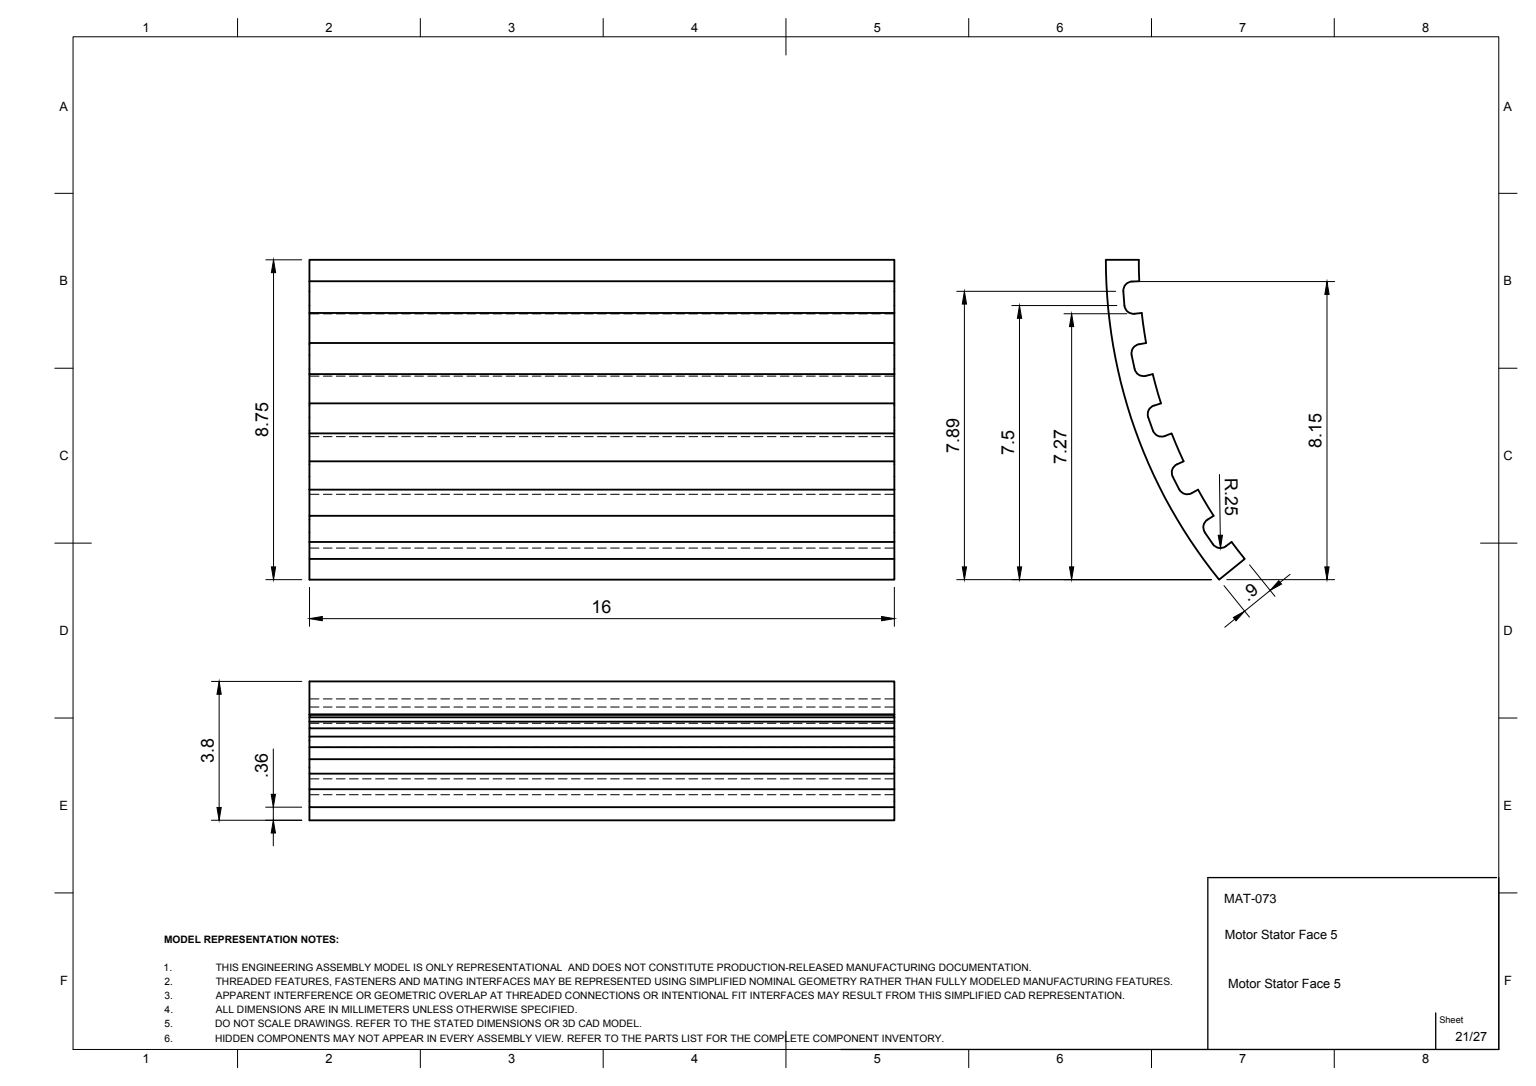
ISO-10303-21;
HEADER;
/* Generated by software containing ST-Developer
 * from STEP Tools, Inc. (www.steptools.com) 
 */

FILE_DESCRIPTION(
/* description */ ('CAx-IF Rec.Pracs.---Representation and Presentation of Product Manufa
cturing Information (PMI)---4.0---2014-10-13'),
/* implementation_level */ '2;1');

FILE_NAME(
/* name */ 'Motor Stator Face 5.step',
/* time_stamp */ '2026-10-24T18:52:33-07:00',
/* author */ (''),
/* organization */ (''),
/* preprocessor_version */ 'ST-DEVELOPER v20.2',
/* originating_system */ 'Autodesk Translation Framework v15.17.0.0',
/* authorisation */ '');

FILE_SCHEMA (('AP242_MANAGED_MODEL_BASED_3D_ENGINEERING_MIM_LF { 1 0 10303 442 2 1 4 }'));
ENDSEC;

DATA;
#10=MECHANICAL_DESIGN_GEOMETRIC_PRESENTATION_REPRESENTATION('',(#436),#34876);
#370=SHAPE_REPRESENTATION_RELATIONSHIP('SRR','None',#35007,#403);
#403=ADVANCED_BREP_SHAPE_REPRESENTATION('',(#469),#34865);
#436=STYLED_ITEM('',(#35165),#469);
#469=MANIFOLD_SOLID_BREP('Motor Stator Face 5',#19576);
#929=PLANE('',#21677);
#930=PLANE('',#21687);
#931=PLANE('',#21697);
#932=PLANE('',#21707);
#933=PLANE('',#21717);
#934=PLANE('',#21718);
#935=PLANE('',#21719);
#936=PLANE('',#21720);
#937=PLANE('',#21721);
#938=PLANE('',#21728);
#939=PLANE('',#21738);
#940=PLANE('',#21741);
#941=PLANE('',#21744);
#942=PLANE('',#21747);
#2176=LINE('',#32962,#3775);
#2177=LINE('',#32965,#3776);
#2178=LINE('',#32970,#3777);
#2179=LINE('',#32976,#3778);
#2180=LINE('',#32980,#3779);
#2181=LINE('',#32982,#3780);
#2182=LINE('',#32983,#3781);
#2183=LINE('',#32989,#3782);
#2184=LINE('',#32992,#3783);
#2185=LINE('',#32997,#3784);
#2186=LINE('',#33003,#3785);
#2187=LINE('',#33007,#3786);
#2188=LINE('',#33009,#3787);
#2189=LINE('',#33010,#3788);
#2190=LINE('',#33016,#3789);
#2191=LINE('',#33019,#3790);
#2192=LINE('',#33024,#3791);
#2193=LINE('',#33030,#3792);
#2194=LINE('',#33034,#3793);
#2195=LINE('',#33036,#3794);
#2196=LINE('',#33037,#3795);
#2197=LINE('',#33043,#3796);
#2198=LINE('',#33046,#3797);
#2199=LINE('',#33051,#3798);
#2200=LINE('',#33057,#3799);
#2201=LINE('',#33061,#3800);
#2202=LINE('',#33063,#3801);
#2203=LINE('',#33064,#3802);
#2204=LINE('',#33070,#3803);
#2205=LINE('',#33073,#3804);
#2206=LINE('',#33078,#3805);
#2207=LINE('',#33084,#3806);
#2208=LINE('',#33088,#3807);
#2209=LINE('',#33090,#3808);
#2210=LINE('',#33091,#3809);
#2211=LINE('',#33094,#3810);
#2212=LINE('',#33096,#3811);
#2213=LINE('',#33097,#3812);
#2214=LINE('',#33100,#3813);
#2215=LINE('',#33102,#3814);
#2216=LINE('',#33103,#3815);
#2217=LINE('',#33106,#3816);
#2218=LINE('',#33108,#3817);
#2219=LINE('',#33109,#3818);
#2220=LINE('',#33112,#3819);
#2221=LINE('',#33114,#3820);
#2222=LINE('',#33115,#3821);
#2223=LINE('',#33120,#3822);
#2224=LINE('',#33127,#3823);
#2225=LINE('',#33131,#3824);
#2226=LINE('',#33136,#3825);
#2227=LINE('',#33141,#3826);
#2228=LINE('',#33144,#3827);
#2229=LINE('',#33147,#3828);
#2230=LINE('',#33152,#3829);
#2231=LINE('',#33153,#3830);
#2232=LINE('',#33157,#3831);
#2233=LINE('',#33159,#3832);
#3775=VECTOR('',#26789,1.);
#3776=VECTOR('',#26792,1.);
#3777=VECTOR('',#26797,1.);
#3778=VECTOR('',#26804,1.);
#3779=VECTOR('',#26809,1.);
#3780=VECTOR('',#26810,1.);
#3781=VECTOR('',#26811,1.);
#3782=VECTOR('',#26816,1.);
#3783=VECTOR('',#26819,1.);
#3784=VECTOR('',#26824,1.);
#3785=VECTOR('',#26831,1.);
#3786=VECTOR('',#26836,1.);
#3787=VECTOR('',#26837,1.);
#3788=VECTOR('',#26838,1.);
#3789=VECTOR('',#26843,1.);
#3790=VECTOR('',#26846,1.);
#3791=VECTOR('',#26851,1.);
#3792=VECTOR('',#26858,1.);
#3793=VECTOR('',#26863,1.);
#3794=VECTOR('',#26864,1.);
#3795=VECTOR('',#26865,1.);
#3796=VECTOR('',#26870,1.);
#3797=VECTOR('',#26873,1.);
#3798=VECTOR('',#26878,1.);
#3799=VECTOR('',#26885,1.);
#3800=VECTOR('',#26890,1.);
#3801=VECTOR('',#26891,1.);
#3802=VECTOR('',#26892,1.);
#3803=VECTOR('',#26897,1.);
#3804=VECTOR('',#26900,1.);
#3805=VECTOR('',#26905,1.);
#3806=VECTOR('',#26912,1.);
#3807=VECTOR('',#26917,1.);
#3808=VECTOR('',#26918,1.);
#3809=VECTOR('',#26919,1.);
#3810=VECTOR('',#26922,1.);
#3811=VECTOR('',#26923,1.);
#3812=VECTOR('',#26924,1.);
#3813=VECTOR('',#26927,1.);
#3814=VECTOR('',#26928,1.);
#3815=VECTOR('',#26929,1.);
#3816=VECTOR('',#26932,1.);
#3817=VECTOR('',#26933,1.);
#3818=VECTOR('',#26934,1.);
#3819=VECTOR('',#26937,1.);
#3820=VECTOR('',#26938,1.);
#3821=VECTOR('',#26939,1.);
#3822=VECTOR('',#26944,1.);
#3823=VECTOR('',#26955,1.);
#3824=VECTOR('',#26958,1.);
#3825=VECTOR('',#26965,1.);
#3826=VECTOR('',#26972,1.);
#3827=VECTOR('',#26975,1.);
#3828=VECTOR('',#26980,1.);
#3829=VECTOR('',#26987,1.);
#3830=VECTOR('',#26988,1.);
#3831=VECTOR('',#26993,1.);
#3832=VECTOR('',#26996,1.);
#4681=CYLINDRICAL_SURFACE('',#21668,0.00025);
#4682=CYLINDRICAL_SURFACE('',#21671,0.01345);
#4683=CYLINDRICAL_SURFACE('',#21674,0.00025);
#4684=CYLINDRICAL_SURFACE('',#21678,0.00025);
#4685=CYLINDRICAL_SURFACE('',#21681,0.01345);
#4686=CYLINDRICAL_SURFACE('',#21684,0.00025);
#4687=CYLINDRICAL_SURFACE('',#21688,0.00025);
#4688=CYLINDRICAL_SURFACE('',#21691,0.01345);
#4689=CYLINDRICAL_SURFACE('',#21694,0.00025);
#4690=CYLINDRICAL_SURFACE('',#21698,0.00025);
#4691=CYLINDRICAL_SURFACE('',#21701,0.01345);
#4692=CYLINDRICAL_SURFACE('',#21704,0.00025);
#4693=CYLINDRICAL_SURFACE('',#21708,0.00025);
#4694=CYLINDRICAL_SURFACE('',#21711,0.01345);
#4695=CYLINDRICAL_SURFACE('',#21714,0.00025);
#4696=CYLINDRICAL_SURFACE('',#21722,0.013);
#4697=CYLINDRICAL_SURFACE('',#21725,0.013);
#4698=CYLINDRICAL_SURFACE('',#21734,0.013);
#4699=CYLINDRICAL_SURFACE('',#21736,0.013);
#4700=CYLINDRICAL_SURFACE('',#21739,0.013);
#4701=CYLINDRICAL_SURFACE('',#21742,0.0139);
#4702=CYLINDRICAL_SURFACE('',#21745,0.013);
#5552=FACE_OUTER_BOUND('',#6679,.T.);
#5553=FACE_OUTER_BOUND('',#6680,.T.);
#5554=FACE_OUTER_BOUND('',#6681,.T.);
#5555=FACE_OUTER_BOUND('',#6682,.T.);
#5556=FACE_OUTER_BOUND('',#6683,.T.);
#5557=FACE_OUTER_BOUND('',#6684,.T.);
#5558=FACE_OUTER_BOUND('',#6685,.T.);
#5559=FACE_OUTER_BOUND('',#6686,.T.);
#5560=FACE_OUTER_BOUND('',#6687,.T.);
#5561=FACE_OUTER_BOUND('',#6688,.T.);
#5562=FACE_OUTER_BOUND('',#6689,.T.);
#5563=FACE_OUTER_BOUND('',#6690,.T.);
#5564=FACE_OUTER_BOUND('',#6691,.T.);
#5565=FACE_OUTER_BOUND('',#6692,.T.);
#5566=FACE_OUTER_BOUND('',#6693,.T.);
#5567=FACE_OUTER_BOUND('',#6694,.T.);
#5568=FACE_OUTER_BOUND('',#6695,.T.);
#5569=FACE_OUTER_BOUND('',#6696,.T.);
#5570=FACE_OUTER_BOUND('',#6697,.T.);
#5571=FACE_OUTER_BOUND('',#6698,.T.);
#5572=FACE_OUTER_BOUND('',#6699,.T.);
#5573=FACE_OUTER_BOUND('',#6700,.T.);
#5574=FACE_OUTER_BOUND('',#6701,.T.);
#5575=FACE_OUTER_BOUND('',#6702,.T.);
#5576=FACE_OUTER_BOUND('',#6703,.T.);
#5577=FACE_OUTER_BOUND('',#6704,.T.);
#5578=FACE_OUTER_BOUND('',#6705,.T.);
#5579=FACE_OUTER_BOUND('',#6706,.T.);
#5580=FACE_OUTER_BOUND('',#6707,.T.);
#5581=FACE_OUTER_BOUND('',#6708,.T.);
#5582=FACE_OUTER_BOUND('',#6709,.T.);
#5583=FACE_OUTER_BOUND('',#6710,.T.);
#5584=FACE_OUTER_BOUND('',#6711,.T.);
#5585=FACE_OUTER_BOUND('',#6712,.T.);
#5586=FACE_OUTER_BOUND('',#6713,.T.);
#5587=FACE_OUTER_BOUND('',#6714,.T.);
#6679=EDGE_LOOP('',(#16904,#16905,#16906,#16907));
#6680=EDGE_LOOP('',(#16908,#16909,#16910,#16911));
#6681=EDGE_LOOP('',(#16912,#16913,#16914,#16915));
#6682=EDGE_LOOP('',(#16916,#16917,#16918,#16919));
#6683=EDGE_LOOP('',(#16920,#16921,#16922,#16923));
#6684=EDGE_LOOP('',(#16924,#16925,#16926,#16927));
#6685=EDGE_LOOP('',(#16928,#16929,#16930,#16931));
#6686=EDGE_LOOP('',(#16932,#16933,#16934,#16935));
#6687=EDGE_LOOP('',(#16936,#16937,#16938,#16939));
#6688=EDGE_LOOP('',(#16940,#16941,#16942,#16943));
#6689=EDGE_LOOP('',(#16944,#16945,#16946,#16947));
#6690=EDGE_LOOP('',(#16948,#16949,#16950,#16951));
#6691=EDGE_LOOP('',(#16952,#16953,#16954,#16955));
#6692=EDGE_LOOP('',(#16956,#16957,#16958,#16959));
#6693=EDGE_LOOP('',(#16960,#16961,#16962,#16963));
#6694=EDGE_LOOP('',(#16964,#16965,#16966,#16967));
#6695=EDGE_LOOP('',(#16968,#16969,#16970,#16971));
#6696=EDGE_LOOP('',(#16972,#16973,#16974,#16975));
#6697=EDGE_LOOP('',(#16976,#16977,#16978,#16979));
#6698=EDGE_LOOP('',(#16980,#16981,#16982,#16983));
#6699=EDGE_LOOP('',(#16984,#16985,#16986,#16987));
#6700=EDGE_LOOP('',(#16988,#16989,#16990,#16991));
#6701=EDGE_LOOP('',(#16992,#16993,#16994,#16995));
#6702=EDGE_LOOP('',(#16996,#16997,#16998,#16999));
#6703=EDGE_LOOP('',(#17000,#17001,#17002,#17003));
#6704=EDGE_LOOP('',(#17004,#17005,#17006,#17007));
#6705=EDGE_LOOP('',(#17008,#17009,#17010,#17011,#17012,#17013,#17014,#17015,
#17016,#17017,#17018,#17019,#17020,#17021,#17022,#17023,#17024,#17025,#17026,
#17027,#17028,#17029,#17030,#17031,#17032,#17033,#17034,#17035,#17036,#17037,
#17038,#17039,#17040,#17041));
#6706=EDGE_LOOP('',(#17042,#17043,#17044,#17045));
#6707=EDGE_LOOP('',(#17046,#17047,#17048,#17049));
#6708=EDGE_LOOP('',(#17050,#17051,#17052,#17053));
#6709=EDGE_LOOP('',(#17054,#17055,#17056,#17057));
#6710=EDGE_LOOP('',(#17058,#17059,#17060,#17061));
#6711=EDGE_LOOP('',(#17062,#17063,#17064,#17065));
#6712=EDGE_LOOP('',(#17066,#17067,#17068,#17069));
#6713=EDGE_LOOP('',(#17070,#17071,#17072,#17073));
#6714=EDGE_LOOP('',(#17074,#17075,#17076,#17077,#17078,#17079,#17080,#17081,
#17082,#17083,#17084,#17085,#17086,#17087,#17088,#17089,#17090,#17091,#17092,
#17093,#17094,#17095,#17096,#17097,#17098,#17099,#17100,#17101,#17102,#17103,
#17104,#17105,#17106,#17107));
#7815=CIRCLE('',#21669,0.000250000000013569);
#7816=CIRCLE('',#21670,0.000250000000013569);
#7817=CIRCLE('',#21672,0.0134500000000125);
#7818=CIRCLE('',#21673,0.0134500000000125);
#7819=CIRCLE('',#21675,0.000250000000013744);
#7820=CIRCLE('',#21676,0.000250000000013744);
#7821=CIRCLE('',#21679,0.000250000000013973);
#7822=CIRCLE('',#21680,0.000250000000013973);
#7823=CIRCLE('',#21682,0.0134500000000115);
#7824=CIRCLE('',#21683,0.0134500000000115);
#7825=CIRCLE('',#21685,0.000250000000014062);
#7826=CIRCLE('',#21686,0.000250000000014062);
#7827=CIRCLE('',#21689,0.000250000000014138);
#7828=CIRCLE('',#21690,0.000250000000014138);
#7829=CIRCLE('',#21692,0.0134500000000103);
#7830=CIRCLE('',#21693,0.0134500000000103);
#7831=CIRCLE('',#21695,0.000250000000014138);
#7832=CIRCLE('',#21696,0.000250000000014138);
#7833=CIRCLE('',#21699,0.000250000000014062);
#7834=CIRCLE('',#21700,0.000250000000014062);
#7835=CIRCLE('',#21702,0.0134500000000109);
#7836=CIRCLE('',#21703,0.0134500000000109);
#7837=CIRCLE('',#21705,0.000250000000013973);
#7838=CIRCLE('',#21706,0.000250000000013973);
#7839=CIRCLE('',#21709,0.000250000000013744);
#7840=CIRCLE('',#21710,0.000250000000013744);
#7841=CIRCLE('',#21712,0.013450000000012);
#7842=CIRCLE('',#21713,0.013450000000012);
#7843=CIRCLE('',#21715,0.000250000000013569);
#7844=CIRCLE('',#21716,0.000250000000013569);
#7845=CIRCLE('',#21723,0.0130000000000128);
#7846=CIRCLE('',#21724,0.0130000000000128);
#7847=CIRCLE('',#21726,0.0130000000000128);
#7848=CIRCLE('',#21727,0.0130000000000128);
#7849=CIRCLE('',#21729,0.0139000000000128);
#7850=CIRCLE('',#21730,0.0130000000000128);
#7851=CIRCLE('',#21731,0.0130000000000128);
#7852=CIRCLE('',#21732,0.0130000000000128);
#7853=CIRCLE('',#21733,0.0130000000000128);
#7854=CIRCLE('',#21735,0.0130000000000128);
#7855=CIRCLE('',#21737,0.0130000000000128);
#7856=CIRCLE('',#21740,0.0130000000000128);
#7857=CIRCLE('',#21743,0.0139000000000128);
#7858=CIRCLE('',#21746,0.0130000000000128);
#9431=VERTEX_POINT('',#32958);
#9432=VERTEX_POINT('',#32959);
#9433=VERTEX_POINT('',#32961);
#9434=VERTEX_POINT('',#32963);
#9435=VERTEX_POINT('',#32967);
#9436=VERTEX_POINT('',#32969);
#9437=VERTEX_POINT('',#32973);
#9438=VERTEX_POINT('',#32975);
#9439=VERTEX_POINT('',#32979);
#9440=VERTEX_POINT('',#32981);
#9441=VERTEX_POINT('',#32985);
#9442=VERTEX_POINT('',#32986);
#9443=VERTEX_POINT('',#32988);
#9444=VERTEX_POINT('',#32990);
#9445=VERTEX_POINT('',#32994);
#9446=VERTEX_POINT('',#32996);
#9447=VERTEX_POINT('',#33000);
#9448=VERTEX_POINT('',#33002);
#9449=VERTEX_POINT('',#33006);
#9450=VERTEX_POINT('',#33008);
#9451=VERTEX_POINT('',#33012);
#9452=VERTEX_POINT('',#33013);
#9453=VERTEX_POINT('',#33015);
#9454=VERTEX_POINT('',#33017);
#9455=VERTEX_POINT('',#33021);
#9456=VERTEX_POINT('',#33023);
#9457=VERTEX_POINT('',#33027);
#9458=VERTEX_POINT('',#33029);
#9459=VERTEX_POINT('',#33033);
#9460=VERTEX_POINT('',#33035);
#9461=VERTEX_POINT('',#33039);
#9462=VERTEX_POINT('',#33040);
#9463=VERTEX_POINT('',#33042);
#9464=VERTEX_POINT('',#33044);
#9465=VERTEX_POINT('',#33048);
#9466=VERTEX_POINT('',#33050);
#9467=VERTEX_POINT('',#33054);
#9468=VERTEX_POINT('',#33056);
#9469=VERTEX_POINT('',#33060);
#9470=VERTEX_POINT('',#33062);
#9471=VERTEX_POINT('',#33066);
#9472=VERTEX_POINT('',#33067);
#9473=VERTEX_POINT('',#33069);
#9474=VERTEX_POINT('',#33071);
#9475=VERTEX_POINT('',#33075);
#9476=VERTEX_POINT('',#33077);
#9477=VERTEX_POINT('',#33081);
#9478=VERTEX_POINT('',#33083);
#9479=VERTEX_POINT('',#33087);
#9480=VERTEX_POINT('',#33089);
#9481=VERTEX_POINT('',#33093);
#9482=VERTEX_POINT('',#33095);
#9483=VERTEX_POINT('',#33099);
#9484=VERTEX_POINT('',#33101);
#9485=VERTEX_POINT('',#33105);
#9486=VERTEX_POINT('',#33107);
#9487=VERTEX_POINT('',#33111);
#9488=VERTEX_POINT('',#33113);
#9489=VERTEX_POINT('',#33117);
#9490=VERTEX_POINT('',#33119);
#9491=VERTEX_POINT('',#33126);
#9492=VERTEX_POINT('',#33128);
#9493=VERTEX_POINT('',#33130);
#9494=VERTEX_POINT('',#33134);
#9495=VERTEX_POINT('',#33139);
#9496=VERTEX_POINT('',#33143);
#9497=VERTEX_POINT('',#33151);
#9498=VERTEX_POINT('',#33155);
#12010=EDGE_CURVE('',#9431,#9432,#7815,.T.);
#12011=EDGE_CURVE('',#9432,#9433,#2176,.T.);
#12012=EDGE_CURVE('',#9433,#9434,#7816,.T.);
#12013=EDGE_CURVE('',#9434,#9431,#2177,.T.);
#12014=EDGE_CURVE('',#9435,#9432,#7817,.T.);
#12015=EDGE_CURVE('',#9436,#9435,#2178,.T.);
#12016=EDGE_CURVE('',#9433,#9436,#7818,.T.);
#12017=EDGE_CURVE('',#9435,#9437,#7819,.T.);
#12018=EDGE_CURVE('',#9437,#9438,#2179,.T.);
#12019=EDGE_CURVE('',#9438,#9436,#7820,.T.);
#12020=EDGE_CURVE('',#9439,#9437,#2180,.T.);
#12021=EDGE_CURVE('',#9440,#9439,#2181,.T.);
#12022=EDGE_CURVE('',#9438,#9440,#2182,.T.);
#12023=EDGE_CURVE('',#9441,#9442,#7821,.T.);
#12024=EDGE_CURVE('',#9442,#9443,#2183,.T.);
#12025=EDGE_CURVE('',#9443,#9444,#7822,.T.);
#12026=EDGE_CURVE('',#9444,#9441,#2184,.T.);
#12027=EDGE_CURVE('',#9445,#9442,#7823,.T.);
#12028=EDGE_CURVE('',#9446,#9445,#2185,.T.);
#12029=EDGE_CURVE('',#9443,#9446,#7824,.T.);
#12030=EDGE_CURVE('',#9445,#9447,#7825,.T.);
#12031=EDGE_CURVE('',#9447,#9448,#2186,.T.);
#12032=EDGE_CURVE('',#9448,#9446,#7826,.T.);
#12033=EDGE_CURVE('',#9449,#9447,#2187,.T.);
#12034=EDGE_CURVE('',#9450,#9449,#2188,.T.);
#12035=EDGE_CURVE('',#9448,#9450,#2189,.T.);
#12036=EDGE_CURVE('',#9451,#9452,#7827,.T.);
#12037=EDGE_CURVE('',#9452,#9453,#2190,.T.);
#12038=EDGE_CURVE('',#9453,#9454,#7828,.T.);
#12039=EDGE_CURVE('',#9454,#9451,#2191,.T.);
#12040=EDGE_CURVE('',#9455,#9452,#7829,.T.);
#12041=EDGE_CURVE('',#9456,#9455,#2192,.T.);
#12042=EDGE_CURVE('',#9453,#9456,#7830,.T.);
#12043=EDGE_CURVE('',#9455,#9457,#7831,.T.);
#12044=EDGE_CURVE('',#9457,#9458,#2193,.T.);
#12045=EDGE_CURVE('',#9458,#9456,#7832,.T.);
#12046=EDGE_CURVE('',#9459,#9457,#2194,.T.);
#12047=EDGE_CURVE('',#9460,#9459,#2195,.T.);
#12048=EDGE_CURVE('',#9458,#9460,#2196,.T.);
#12049=EDGE_CURVE('',#9461,#9462,#7833,.T.);
#12050=EDGE_CURVE('',#9462,#9463,#2197,.T.);
#12051=EDGE_CURVE('',#9463,#9464,#7834,.T.);
#12052=EDGE_CURVE('',#9464,#9461,#2198,.T.);
#12053=EDGE_CURVE('',#9465,#9462,#7835,.T.);
#12054=EDGE_CURVE('',#9466,#9465,#2199,.T.);
#12055=EDGE_CURVE('',#9463,#9466,#7836,.T.);
#12056=EDGE_CURVE('',#9465,#9467,#7837,.T.);
#12057=EDGE_CURVE('',#9467,#9468,#2200,.T.);
#12058=EDGE_CURVE('',#9468,#9466,#7838,.T.);
#12059=EDGE_CURVE('',#9469,#9467,#2201,.T.);
#12060=EDGE_CURVE('',#9470,#9469,#2202,.T.);
#12061=EDGE_CURVE('',#9468,#9470,#2203,.T.);
#12062=EDGE_CURVE('',#9471,#9472,#7839,.T.);
#12063=EDGE_CURVE('',#9472,#9473,#2204,.T.);
#12064=EDGE_CURVE('',#9473,#9474,#7840,.T.);
#12065=EDGE_CURVE('',#9474,#9471,#2205,.T.);
#12066=EDGE_CURVE('',#9475,#9472,#7841,.T.);
#12067=EDGE_CURVE('',#9476,#9475,#2206,.T.);
#12068=EDGE_CURVE('',#9473,#9476,#7842,.T.);
#12069=EDGE_CURVE('',#9475,#9477,#7843,.T.);
#12070=EDGE_CURVE('',#9477,#9478,#2207,.T.);
#12071=EDGE_CURVE('',#9478,#9476,#7844,.T.);
#12072=EDGE_CURVE('',#9479,#9477,#2208,.T.);
#12073=EDGE_CURVE('',#9480,#9479,#2209,.T.);
#12074=EDGE_CURVE('',#9478,#9480,#2210,.T.);
#12075=EDGE_CURVE('',#9481,#9474,#2211,.T.);
#12076=EDGE_CURVE('',#9482,#9481,#2212,.T.);
#12077=EDGE_CURVE('',#9471,#9482,#2213,.T.);
#12078=EDGE_CURVE('',#9483,#9464,#2214,.T.);
#12079=EDGE_CURVE('',#9484,#9483,#2215,.T.);
#12080=EDGE_CURVE('',#9461,#9484,#2216,.T.);
#12081=EDGE_CURVE('',#9485,#9444,#2217,.T.);
#12082=EDGE_CURVE('',#9486,#9485,#2218,.T.);
#12083=EDGE_CURVE('',#9441,#9486,#2219,.T.);
#12084=EDGE_CURVE('',#9487,#9434,#2220,.T.);
#12085=EDGE_CURVE('',#9488,#9487,#2221,.T.);
#12086=EDGE_CURVE('',#9431,#9488,#2222,.T.);
#12087=EDGE_CURVE('',#9489,#9479,#7845,.T.);
#12088=EDGE_CURVE('',#9489,#9490,#2223,.T.);
#12089=EDGE_CURVE('',#9480,#9490,#7846,.T.);
#12090=EDGE_CURVE('',#9460,#9483,#7847,.T.);
#12091=EDGE_CURVE('',#9484,#9459,#7848,.T.);
#12092=EDGE_CURVE('',#9490,#9491,#2224,.T.);
#12093=EDGE_CURVE('',#9491,#9492,#7849,.T.);
#12094=EDGE_CURVE('',#9492,#9493,#2225,.T.);
#12095=EDGE_CURVE('',#9493,#9487,#7850,.T.);
#12096=EDGE_CURVE('',#9440,#9485,#7851,.T.);
#12097=EDGE_CURVE('',#9450,#9494,#7852,.T.);
#12098=EDGE_CURVE('',#9494,#9454,#2226,.T.);
#12099=EDGE_CURVE('',#9470,#9481,#7853,.T.);
#12100=EDGE_CURVE('',#9495,#9449,#7854,.T.);
#12101=EDGE_CURVE('',#9495,#9494,#2227,.T.);
#12102=EDGE_CURVE('',#9493,#9496,#2228,.T.);
#12103=EDGE_CURVE('',#9488,#9496,#7855,.T.);
#12104=EDGE_CURVE('',#9451,#9495,#2229,.T.);
#12105=EDGE_CURVE('',#9482,#9469,#7856,.T.);
#12106=EDGE_CURVE('',#9497,#9489,#2230,.T.);
#12107=EDGE_CURVE('',#9491,#9497,#2231,.T.);
#12108=EDGE_CURVE('',#9498,#9497,#7857,.T.);
#12109=EDGE_CURVE('',#9492,#9498,#2232,.T.);
#12110=EDGE_CURVE('',#9496,#9498,#2233,.T.);
#12111=EDGE_CURVE('',#9486,#9439,#7858,.T.);
#16904=ORIENTED_EDGE('',*,*,#12010,.T.);
#16905=ORIENTED_EDGE('',*,*,#12011,.T.);
#16906=ORIENTED_EDGE('',*,*,#12012,.T.);
#16907=ORIENTED_EDGE('',*,*,#12013,.T.);
#16908=ORIENTED_EDGE('',*,*,#12011,.F.);
#16909=ORIENTED_EDGE('',*,*,#12014,.F.);
#16910=ORIENTED_EDGE('',*,*,#12015,.F.);
#16911=ORIENTED_EDGE('',*,*,#12016,.F.);
#16912=ORIENTED_EDGE('',*,*,#12017,.T.);
#16913=ORIENTED_EDGE('',*,*,#12018,.T.);
#16914=ORIENTED_EDGE('',*,*,#12019,.T.);
#16915=ORIENTED_EDGE('',*,*,#12015,.T.);
#16916=ORIENTED_EDGE('',*,*,#12018,.F.);
#16917=ORIENTED_EDGE('',*,*,#12020,.F.);
#16918=ORIENTED_EDGE('',*,*,#12021,.F.);
#16919=ORIENTED_EDGE('',*,*,#12022,.F.);
#16920=ORIENTED_EDGE('',*,*,#12023,.T.);
#16921=ORIENTED_EDGE('',*,*,#12024,.T.);
#16922=ORIENTED_EDGE('',*,*,#12025,.T.);
#16923=ORIENTED_EDGE('',*,*,#12026,.T.);
#16924=ORIENTED_EDGE('',*,*,#12024,.F.);
#16925=ORIENTED_EDGE('',*,*,#12027,.F.);
#16926=ORIENTED_EDGE('',*,*,#12028,.F.);
#16927=ORIENTED_EDGE('',*,*,#12029,.F.);
#16928=ORIENTED_EDGE('',*,*,#12030,.T.);
#16929=ORIENTED_EDGE('',*,*,#12031,.T.);
#16930=ORIENTED_EDGE('',*,*,#12032,.T.);
#16931=ORIENTED_EDGE('',*,*,#12028,.T.);
#16932=ORIENTED_EDGE('',*,*,#12031,.F.);
#16933=ORIENTED_EDGE('',*,*,#12033,.F.);
#16934=ORIENTED_EDGE('',*,*,#12034,.F.);
#16935=ORIENTED_EDGE('',*,*,#12035,.F.);
#16936=ORIENTED_EDGE('',*,*,#12036,.T.);
#16937=ORIENTED_EDGE('',*,*,#12037,.T.);
#16938=ORIENTED_EDGE('',*,*,#12038,.T.);
#16939=ORIENTED_EDGE('',*,*,#12039,.T.);
#16940=ORIENTED_EDGE('',*,*,#12037,.F.);
#16941=ORIENTED_EDGE('',*,*,#12040,.F.);
#16942=ORIENTED_EDGE('',*,*,#12041,.F.);
#16943=ORIENTED_EDGE('',*,*,#12042,.F.);
#16944=ORIENTED_EDGE('',*,*,#12043,.T.);
#16945=ORIENTED_EDGE('',*,*,#12044,.T.);
#16946=ORIENTED_EDGE('',*,*,#12045,.T.);
#16947=ORIENTED_EDGE('',*,*,#12041,.T.);
#16948=ORIENTED_EDGE('',*,*,#12044,.F.);
#16949=ORIENTED_EDGE('',*,*,#12046,.F.);
#16950=ORIENTED_EDGE('',*,*,#12047,.F.);
#16951=ORIENTED_EDGE('',*,*,#12048,.F.);
#16952=ORIENTED_EDGE('',*,*,#12049,.T.);
#16953=ORIENTED_EDGE('',*,*,#12050,.T.);
#16954=ORIENTED_EDGE('',*,*,#12051,.T.);
#16955=ORIENTED_EDGE('',*,*,#12052,.T.);
#16956=ORIENTED_EDGE('',*,*,#12050,.F.);
#16957=ORIENTED_EDGE('',*,*,#12053,.F.);
#16958=ORIENTED_EDGE('',*,*,#12054,.F.);
#16959=ORIENTED_EDGE('',*,*,#12055,.F.);
#16960=ORIENTED_EDGE('',*,*,#12056,.T.);
#16961=ORIENTED_EDGE('',*,*,#12057,.T.);
#16962=ORIENTED_EDGE('',*,*,#12058,.T.);
#16963=ORIENTED_EDGE('',*,*,#12054,.T.);
#16964=ORIENTED_EDGE('',*,*,#12057,.F.);
#16965=ORIENTED_EDGE('',*,*,#12059,.F.);
#16966=ORIENTED_EDGE('',*,*,#12060,.F.);
#16967=ORIENTED_EDGE('',*,*,#12061,.F.);
#16968=ORIENTED_EDGE('',*,*,#12062,.T.);
#16969=ORIENTED_EDGE('',*,*,#12063,.T.);
#16970=ORIENTED_EDGE('',*,*,#12064,.T.);
#16971=ORIENTED_EDGE('',*,*,#12065,.T.);
#16972=ORIENTED_EDGE('',*,*,#12063,.F.);
#16973=ORIENTED_EDGE('',*,*,#12066,.F.);
#16974=ORIENTED_EDGE('',*,*,#12067,.F.);
#16975=ORIENTED_EDGE('',*,*,#12068,.F.);
#16976=ORIENTED_EDGE('',*,*,#12069,.T.);
#16977=ORIENTED_EDGE('',*,*,#12070,.T.);
#16978=ORIENTED_EDGE('',*,*,#12071,.T.);
#16979=ORIENTED_EDGE('',*,*,#12067,.T.);
#16980=ORIENTED_EDGE('',*,*,#12070,.F.);
#16981=ORIENTED_EDGE('',*,*,#12072,.F.);
#16982=ORIENTED_EDGE('',*,*,#12073,.F.);
#16983=ORIENTED_EDGE('',*,*,#12074,.F.);
#16984=ORIENTED_EDGE('',*,*,#12065,.F.);
#16985=ORIENTED_EDGE('',*,*,#12075,.F.);
#16986=ORIENTED_EDGE('',*,*,#12076,.F.);
#16987=ORIENTED_EDGE('',*,*,#12077,.F.);
#16988=ORIENTED_EDGE('',*,*,#12052,.F.);
#16989=ORIENTED_EDGE('',*,*,#12078,.F.);
#16990=ORIENTED_EDGE('',*,*,#12079,.F.);
#16991=ORIENTED_EDGE('',*,*,#12080,.F.);
#16992=ORIENTED_EDGE('',*,*,#12026,.F.);
#16993=ORIENTED_EDGE('',*,*,#12081,.F.);
#16994=ORIENTED_EDGE('',*,*,#12082,.F.);
#16995=ORIENTED_EDGE('',*,*,#12083,.F.);
#16996=ORIENTED_EDGE('',*,*,#12013,.F.);
#16997=ORIENTED_EDGE('',*,*,#12084,.F.);
#16998=ORIENTED_EDGE('',*,*,#12085,.F.);
#16999=ORIENTED_EDGE('',*,*,#12086,.F.);
#17000=ORIENTED_EDGE('',*,*,#12073,.T.);
#17001=ORIENTED_EDGE('',*,*,#12087,.F.);
#17002=ORIENTED_EDGE('',*,*,#12088,.T.);
#17003=ORIENTED_EDGE('',*,*,#12089,.F.);
#17004=ORIENTED_EDGE('',*,*,#12079,.T.);
#17005=ORIENTED_EDGE('',*,*,#12090,.F.);
#17006=ORIENTED_EDGE('',*,*,#12047,.T.);
#17007=ORIENTED_EDGE('',*,*,#12091,.F.);
#17008=ORIENTED_EDGE('',*,*,#12075,.T.);
#17009=ORIENTED_EDGE('',*,*,#12064,.F.);
#17010=ORIENTED_EDGE('',*,*,#12068,.T.);
#17011=ORIENTED_EDGE('',*,*,#12071,.F.);
#17012=ORIENTED_EDGE('',*,*,#12074,.T.);
#17013=ORIENTED_EDGE('',*,*,#12089,.T.);
#17014=ORIENTED_EDGE('',*,*,#12092,.T.);
#17015=ORIENTED_EDGE('',*,*,#12093,.T.);
#17016=ORIENTED_EDGE('',*,*,#12094,.T.);
#17017=ORIENTED_EDGE('',*,*,#12095,.T.);
#17018=ORIENTED_EDGE('',*,*,#12084,.T.);
#17019=ORIENTED_EDGE('',*,*,#12012,.F.);
#17020=ORIENTED_EDGE('',*,*,#12016,.T.);
#17021=ORIENTED_EDGE('',*,*,#12019,.F.);
#17022=ORIENTED_EDGE('',*,*,#12022,.T.);
#17023=ORIENTED_EDGE('',*,*,#12096,.T.);
#17024=ORIENTED_EDGE('',*,*,#12081,.T.);
#17025=ORIENTED_EDGE('',*,*,#12025,.F.);
#17026=ORIENTED_EDGE('',*,*,#12029,.T.);
#17027=ORIENTED_EDGE('',*,*,#12032,.F.);
#17028=ORIENTED_EDGE('',*,*,#12035,.T.);
#17029=ORIENTED_EDGE('',*,*,#12097,.T.);
#17030=ORIENTED_EDGE('',*,*,#12098,.T.);
#17031=ORIENTED_EDGE('',*,*,#12038,.F.);
#17032=ORIENTED_EDGE('',*,*,#12042,.T.);
#17033=ORIENTED_EDGE('',*,*,#12045,.F.);
#17034=ORIENTED_EDGE('',*,*,#12048,.T.);
#17035=ORIENTED_EDGE('',*,*,#12090,.T.);
#17036=ORIENTED_EDGE('',*,*,#12078,.T.);
#17037=ORIENTED_EDGE('',*,*,#12051,.F.);
#17038=ORIENTED_EDGE('',*,*,#12055,.T.);
#17039=ORIENTED_EDGE('',*,*,#12058,.F.);
#17040=ORIENTED_EDGE('',*,*,#12061,.T.);
#17041=ORIENTED_EDGE('',*,*,#12099,.T.);
#17042=ORIENTED_EDGE('',*,*,#12034,.T.);
#17043=ORIENTED_EDGE('',*,*,#12100,.F.);
#17044=ORIENTED_EDGE('',*,*,#12101,.T.);
#17045=ORIENTED_EDGE('',*,*,#12097,.F.);
#17046=ORIENTED_EDGE('',*,*,#12085,.T.);
#17047=ORIENTED_EDGE('',*,*,#12095,.F.);
#17048=ORIENTED_EDGE('',*,*,#12102,.T.);
#17049=ORIENTED_EDGE('',*,*,#12103,.F.);
#17050=ORIENTED_EDGE('',*,*,#12039,.F.);
#17051=ORIENTED_EDGE('',*,*,#12098,.F.);
#17052=ORIENTED_EDGE('',*,*,#12101,.F.);
#17053=ORIENTED_EDGE('',*,*,#12104,.F.);
#17054=ORIENTED_EDGE('',*,*,#12076,.T.);
#17055=ORIENTED_EDGE('',*,*,#12099,.F.);
#17056=ORIENTED_EDGE('',*,*,#12060,.T.);
#17057=ORIENTED_EDGE('',*,*,#12105,.F.);
#17058=ORIENTED_EDGE('',*,*,#12088,.F.);
#17059=ORIENTED_EDGE('',*,*,#12106,.F.);
#17060=ORIENTED_EDGE('',*,*,#12107,.F.);
#17061=ORIENTED_EDGE('',*,*,#12092,.F.);
#17062=ORIENTED_EDGE('',*,*,#12107,.T.);
#17063=ORIENTED_EDGE('',*,*,#12108,.F.);
#17064=ORIENTED_EDGE('',*,*,#12109,.F.);
#17065=ORIENTED_EDGE('',*,*,#12093,.F.);
#17066=ORIENTED_EDGE('',*,*,#12109,.T.);
#17067=ORIENTED_EDGE('',*,*,#12110,.F.);
#17068=ORIENTED_EDGE('',*,*,#12102,.F.);
#17069=ORIENTED_EDGE('',*,*,#12094,.F.);
#17070=ORIENTED_EDGE('',*,*,#12082,.T.);
#17071=ORIENTED_EDGE('',*,*,#12096,.F.);
#17072=ORIENTED_EDGE('',*,*,#12021,.T.);
#17073=ORIENTED_EDGE('',*,*,#12111,.F.);
#17074=ORIENTED_EDGE('',*,*,#12077,.T.);
#17075=ORIENTED_EDGE('',*,*,#12105,.T.);
#17076=ORIENTED_EDGE('',*,*,#12059,.T.);
#17077=ORIENTED_EDGE('',*,*,#12056,.F.);
#17078=ORIENTED_EDGE('',*,*,#12053,.T.);
#17079=ORIENTED_EDGE('',*,*,#12049,.F.);
#17080=ORIENTED_EDGE('',*,*,#12080,.T.);
#17081=ORIENTED_EDGE('',*,*,#12091,.T.);
#17082=ORIENTED_EDGE('',*,*,#12046,.T.);
#17083=ORIENTED_EDGE('',*,*,#12043,.F.);
#17084=ORIENTED_EDGE('',*,*,#12040,.T.);
#17085=ORIENTED_EDGE('',*,*,#12036,.F.);
#17086=ORIENTED_EDGE('',*,*,#12104,.T.);
#17087=ORIENTED_EDGE('',*,*,#12100,.T.);
#17088=ORIENTED_EDGE('',*,*,#12033,.T.);
#17089=ORIENTED_EDGE('',*,*,#12030,.F.);
#17090=ORIENTED_EDGE('',*,*,#12027,.T.);
#17091=ORIENTED_EDGE('',*,*,#12023,.F.);
#17092=ORIENTED_EDGE('',*,*,#12083,.T.);
#17093=ORIENTED_EDGE('',*,*,#12111,.T.);
#17094=ORIENTED_EDGE('',*,*,#12020,.T.);
#17095=ORIENTED_EDGE('',*,*,#12017,.F.);
#17096=ORIENTED_EDGE('',*,*,#12014,.T.);
#17097=ORIENTED_EDGE('',*,*,#12010,.F.);
#17098=ORIENTED_EDGE('',*,*,#12086,.T.);
#17099=ORIENTED_EDGE('',*,*,#12103,.T.);
#17100=ORIENTED_EDGE('',*,*,#12110,.T.);
#17101=ORIENTED_EDGE('',*,*,#12108,.T.);
#17102=ORIENTED_EDGE('',*,*,#12106,.T.);
#17103=ORIENTED_EDGE('',*,*,#12087,.T.);
#17104=ORIENTED_EDGE('',*,*,#12072,.T.);
#17105=ORIENTED_EDGE('',*,*,#12069,.F.);
#17106=ORIENTED_EDGE('',*,*,#12066,.T.);
#17107=ORIENTED_EDGE('',*,*,#12062,.F.);
#19268=ADVANCED_FACE('',(#5552),#4681,.F.);
#19269=ADVANCED_FACE('',(#5553),#4682,.F.);
#19270=ADVANCED_FACE('',(#5554),#4683,.F.);
#19271=ADVANCED_FACE('',(#5555),#929,.F.);
#19272=ADVANCED_FACE('',(#5556),#4684,.F.);
#19273=ADVANCED_FACE('',(#5557),#4685,.F.);
#19274=ADVANCED_FACE('',(#5558),#4686,.F.);
#19275=ADVANCED_FACE('',(#5559),#930,.F.);
#19276=ADVANCED_FACE('',(#5560),#4687,.F.);
#19277=ADVANCED_FACE('',(#5561),#4688,.F.);
#19278=ADVANCED_FACE('',(#5562),#4689,.F.);
#19279=ADVANCED_FACE('',(#5563),#931,.F.);
#19280=ADVANCED_FACE('',(#5564),#4690,.F.);
#19281=ADVANCED_FACE('',(#5565),#4691,.F.);
#19282=ADVANCED_FACE('',(#5566),#4692,.F.);
#19283=ADVANCED_FACE('',(#5567),#932,.F.);
#19284=ADVANCED_FACE('',(#5568),#4693,.F.);
#19285=ADVANCED_FACE('',(#5569),#4694,.F.);
#19286=ADVANCED_FACE('',(#5570),#4695,.F.);
#19287=ADVANCED_FACE('',(#5571),#933,.F.);
#19288=ADVANCED_FACE('',(#5572),#934,.F.);
#19289=ADVANCED_FACE('',(#5573),#935,.F.);
#19290=ADVANCED_FACE('',(#5574),#936,.F.);
#19291=ADVANCED_FACE('',(#5575),#937,.F.);
#19292=ADVANCED_FACE('',(#5576),#4696,.F.);
#19293=ADVANCED_FACE('',(#5577),#4697,.F.);
#19294=ADVANCED_FACE('',(#5578),#938,.F.);
#19295=ADVANCED_FACE('',(#5579),#4698,.F.);
#19296=ADVANCED_FACE('',(#5580),#4699,.F.);
#19297=ADVANCED_FACE('',(#5581),#939,.F.);
#19298=ADVANCED_FACE('',(#5582),#4700,.F.);
#19299=ADVANCED_FACE('',(#5583),#940,.T.);
#19300=ADVANCED_FACE('',(#5584),#4701,.T.);
#19301=ADVANCED_FACE('',(#5585),#941,.T.);
#19302=ADVANCED_FACE('',(#5586),#4702,.F.);
#19303=ADVANCED_FACE('',(#5587),#942,.T.);
#19576=CLOSED_SHELL('',(#19268,#19269,#19270,#19271,#19272,#19273,#19274,
#19275,#19276,#19277,#19278,#19279,#19280,#19281,#19282,#19283,#19284,#19285,
#19286,#19287,#19288,#19289,#19290,#19291,#19292,#19293,#19294,#19295,#19296,
#19297,#19298,#19299,#19300,#19301,#19302,#19303));
#21667=AXIS2_PLACEMENT_3D('',#32956,#26783,#26784);
#21668=AXIS2_PLACEMENT_3D('',#32957,#26785,#26786);
#21669=AXIS2_PLACEMENT_3D('',#32960,#26787,#26788);
#21670=AXIS2_PLACEMENT_3D('',#32964,#26790,#26791);
#21671=AXIS2_PLACEMENT_3D('',#32966,#26793,#26794);
#21672=AXIS2_PLACEMENT_3D('',#32968,#26795,#26796);
#21673=AXIS2_PLACEMENT_3D('',#32971,#26798,#26799);
#21674=AXIS2_PLACEMENT_3D('',#32972,#26800,#26801);
#21675=AXIS2_PLACEMENT_3D('',#32974,#26802,#26803);
#21676=AXIS2_PLACEMENT_3D('',#32977,#26805,#26806);
#21677=AXIS2_PLACEMENT_3D('',#32978,#26807,#26808);
#21678=AXIS2_PLACEMENT_3D('',#32984,#26812,#26813);
#21679=AXIS2_PLACEMENT_3D('',#32987,#26814,#26815);
#21680=AXIS2_PLACEMENT_3D('',#32991,#26817,#26818);
#21681=AXIS2_PLACEMENT_3D('',#32993,#26820,#26821);
#21682=AXIS2_PLACEMENT_3D('',#32995,#26822,#26823);
#21683=AXIS2_PLACEMENT_3D('',#32998,#26825,#26826);
#21684=AXIS2_PLACEMENT_3D('',#32999,#26827,#26828);
#21685=AXIS2_PLACEMENT_3D('',#33001,#26829,#26830);
#21686=AXIS2_PLACEMENT_3D('',#33004,#26832,#26833);
#21687=AXIS2_PLACEMENT_3D('',#33005,#26834,#26835);
#21688=AXIS2_PLACEMENT_3D('',#33011,#26839,#26840);
#21689=AXIS2_PLACEMENT_3D('',#33014,#26841,#26842);
#21690=AXIS2_PLACEMENT_3D('',#33018,#26844,#26845);
#21691=AXIS2_PLACEMENT_3D('',#33020,#26847,#26848);
#21692=AXIS2_PLACEMENT_3D('',#33022,#26849,#26850);
#21693=AXIS2_PLACEMENT_3D('',#33025,#26852,#26853);
#21694=AXIS2_PLACEMENT_3D('',#33026,#26854,#26855);
#21695=AXIS2_PLACEMENT_3D('',#33028,#26856,#26857);
#21696=AXIS2_PLACEMENT_3D('',#33031,#26859,#26860);
#21697=AXIS2_PLACEMENT_3D('',#33032,#26861,#26862);
#21698=AXIS2_PLACEMENT_3D('',#33038,#26866,#26867);
#21699=AXIS2_PLACEMENT_3D('',#33041,#26868,#26869);
#21700=AXIS2_PLACEMENT_3D('',#33045,#26871,#26872);
#21701=AXIS2_PLACEMENT_3D('',#33047,#26874,#26875);
#21702=AXIS2_PLACEMENT_3D('',#33049,#26876,#26877);
#21703=AXIS2_PLACEMENT_3D('',#33052,#26879,#26880);
#21704=AXIS2_PLACEMENT_3D('',#33053,#26881,#26882);
#21705=AXIS2_PLACEMENT_3D('',#33055,#26883,#26884);
#21706=AXIS2_PLACEMENT_3D('',#33058,#26886,#26887);
#21707=AXIS2_PLACEMENT_3D('',#33059,#26888,#26889);
#21708=AXIS2_PLACEMENT_3D('',#33065,#26893,#26894);
#21709=AXIS2_PLACEMENT_3D('',#33068,#26895,#26896);
#21710=AXIS2_PLACEMENT_3D('',#33072,#26898,#26899);
#21711=AXIS2_PLACEMENT_3D('',#33074,#26901,#26902);
#21712=AXIS2_PLACEMENT_3D('',#33076,#26903,#26904);
#21713=AXIS2_PLACEMENT_3D('',#33079,#26906,#26907);
#21714=AXIS2_PLACEMENT_3D('',#33080,#26908,#26909);
#21715=AXIS2_PLACEMENT_3D('',#33082,#26910,#26911);
#21716=AXIS2_PLACEMENT_3D('',#33085,#26913,#26914);
#21717=AXIS2_PLACEMENT_3D('',#33086,#26915,#26916);
#21718=AXIS2_PLACEMENT_3D('',#33092,#26920,#26921);
#21719=AXIS2_PLACEMENT_3D('',#33098,#26925,#26926);
#21720=AXIS2_PLACEMENT_3D('',#33104,#26930,#26931);
#21721=AXIS2_PLACEMENT_3D('',#33110,#26935,#26936);
#21722=AXIS2_PLACEMENT_3D('',#33116,#26940,#26941);
#21723=AXIS2_PLACEMENT_3D('',#33118,#26942,#26943);
#21724=AXIS2_PLACEMENT_3D('',#33121,#26945,#26946);
#21725=AXIS2_PLACEMENT_3D('',#33122,#26947,#26948);
#21726=AXIS2_PLACEMENT_3D('',#33123,#26949,#26950);
#21727=AXIS2_PLACEMENT_3D('',#33124,#26951,#26952);
#21728=AXIS2_PLACEMENT_3D('',#33125,#26953,#26954);
#21729=AXIS2_PLACEMENT_3D('',#33129,#26956,#26957);
#21730=AXIS2_PLACEMENT_3D('',#33132,#26959,#26960);
#21731=AXIS2_PLACEMENT_3D('',#33133,#26961,#26962);
#21732=AXIS2_PLACEMENT_3D('',#33135,#26963,#26964);
#21733=AXIS2_PLACEMENT_3D('',#33137,#26966,#26967);
#21734=AXIS2_PLACEMENT_3D('',#33138,#26968,#26969);
#21735=AXIS2_PLACEMENT_3D('',#33140,#26970,#26971);
#21736=AXIS2_PLACEMENT_3D('',#33142,#26973,#26974);
#21737=AXIS2_PLACEMENT_3D('',#33145,#26976,#26977);
#21738=AXIS2_PLACEMENT_3D('',#33146,#26978,#26979);
#21739=AXIS2_PLACEMENT_3D('',#33148,#26981,#26982);
#21740=AXIS2_PLACEMENT_3D('',#33149,#26983,#26984);
#21741=AXIS2_PLACEMENT_3D('',#33150,#26985,#26986);
#21742=AXIS2_PLACEMENT_3D('',#33154,#26989,#26990);
#21743=AXIS2_PLACEMENT_3D('',#33156,#26991,#26992);
#21744=AXIS2_PLACEMENT_3D('',#33158,#26994,#26995);
#21745=AXIS2_PLACEMENT_3D('',#33160,#26997,#26998);
#21746=AXIS2_PLACEMENT_3D('',#33161,#26999,#27000);
#21747=AXIS2_PLACEMENT_3D('',#33162,#27001,#27002);
#26783=DIRECTION('axis',(0.,0.,1.));
#26784=DIRECTION('refdir',(1.,0.,0.));
#26785=DIRECTION('center_axis',(0.,-1.,0.));
#26786=DIRECTION('ref_axis',(0.479079334165908,0.,0.877771605587211));
#26787=DIRECTION('center_axis',(0.,1.,0.));
#26788=DIRECTION('ref_axis',(0.479079334179906,0.,0.877771605579571));
#26789=DIRECTION('',(0.,-1.,0.));
#26790=DIRECTION('center_axis',(0.,-1.,0.));
#26791=DIRECTION('ref_axis',(0.479079334179906,0.,0.877771605579571));
#26792=DIRECTION('',(0.,1.,0.));
#26793=DIRECTION('center_axis',(0.,-1.,0.));
#26794=DIRECTION('ref_axis',(0.956725679001188,0.,0.290991366091359));
#26795=DIRECTION('center_axis',(0.,-1.,0.));
#26796=DIRECTION('ref_axis',(0.956725679001044,0.,0.290991366091832));
#26797=DIRECTION('',(0.,1.,0.));
#26798=DIRECTION('center_axis',(0.,1.,0.));
#26799=DIRECTION('ref_axis',(0.956725679001044,0.,0.290991366091832));
#26800=DIRECTION('center_axis',(0.,-1.,0.));
#26801=DIRECTION('ref_axis',(0.853780676609416,0.,-0.520632842076226));
#26802=DIRECTION('center_axis',(0.,1.,0.));
#26803=DIRECTION('ref_axis',(0.853780676602478,0.,-0.520632842087603));
#26804=DIRECTION('',(0.,-1.,0.));
#26805=DIRECTION('center_axis',(0.,-1.,0.));
#26806=DIRECTION('ref_axis',(0.853780676602478,0.,-0.520632842087603));
#26807=DIRECTION('center_axis',(0.22635692418354,0.,-0.974044425513625));
#26808=DIRECTION('ref_axis',(0.,-1.,0.));
#26809=DIRECTION('',(0.974044425513455,0.,0.226356924184268));
#26810=DIRECTION('',(0.,1.,0.));
#26811=DIRECTION('',(-0.974044425513455,0.,-0.226356924184268));
#26812=DIRECTION('center_axis',(0.,-1.,0.));
#26813=DIRECTION('ref_axis',(0.589552929365364,0.,0.80772974655928));
#26814=DIRECTION('center_axis',(0.,1.,0.));
#26815=DIRECTION('ref_axis',(0.589552929372413,0.,0.807729746554134));
#26816=DIRECTION('',(0.,-1.,0.));
#26817=DIRECTION('center_axis',(0.,-1.,0.));
#26818=DIRECTION('ref_axis',(0.589552929372413,0.,0.807729746554134));
#26819=DIRECTION('',(0.,1.,0.));
#26820=DIRECTION('center_axis',(0.,-1.,0.));
#26821=DIRECTION('ref_axis',(0.986522753174914,0.,0.163624134736254));
#26822=DIRECTION('center_axis',(0.,-1.,0.));
#26823=DIRECTION('ref_axis',(0.986522753174814,0.,0.163624134736857));
#26824=DIRECTION('',(0.,1.,0.));
#26825=DIRECTION('center_axis',(0.,1.,0.));
#26826=DIRECTION('ref_axis',(0.986522753174814,0.,0.163624134736857));
#26827=DIRECTION('center_axis',(0.,-1.,0.));
#26828=DIRECTION('ref_axis',(0.778520242143747,0.,-0.627619496647803));
#26829=DIRECTION('center_axis',(0.,1.,0.));
#26830=DIRECTION('ref_axis',(0.778520242139959,0.,-0.627619496652502));
#26831=DIRECTION('',(0.,-1.,0.));
#26832=DIRECTION('center_axis',(0.,-1.,0.));
#26833=DIRECTION('ref_axis',(0.778520242139959,0.,-0.627619496652502));
#26834=DIRECTION('center_axis',(0.0972820994026908,0.,-0.995256847821609));
#26835=DIRECTION('ref_axis',(0.,-1.,0.));
#26836=DIRECTION('',(0.995256847821521,0.,0.0972820994035846));
#26837=DIRECTION('',(0.,1.,0.));
#26838=DIRECTION('',(-0.995256847821521,0.,-0.0972820994035846));
#26839=DIRECTION('center_axis',(0.,-1.,0.));
#26840=DIRECTION('ref_axis',(0.689939110488415,0.,0.723867407622732));
#26841=DIRECTION('center_axis',(0.,1.,0.));
#26842=DIRECTION('ref_axis',(0.689939110489398,0.,0.723867407621795));
#26843=DIRECTION('',(0.,-1.,0.));
#26844=DIRECTION('center_axis',(0.,-1.,0.));
#26845=DIRECTION('ref_axis',(0.689939110489398,0.,0.723867407621795));
#26846=DIRECTION('',(0.,1.,0.));
#26847=DIRECTION('center_axis',(0.,-1.,0.));
#26848=DIRECTION('ref_axis',(0.999440149526036,0.,0.033457249070632));
#26849=DIRECTION('center_axis',(0.,-1.,0.));
#26850=DIRECTION('ref_axis',(0.999440149526012,0.,0.0334572490713498));
#26851=DIRECTION('',(0.,1.,0.));
#26852=DIRECTION('center_axis',(0.,1.,0.));
#26853=DIRECTION('ref_axis',(0.999440149526012,0.,0.0334572490713498));
#26854=DIRECTION('center_axis',(0.,-1.,0.));
#26855=DIRECTION('ref_axis',(0.689939110488415,0.,-0.723867407622732));
#26856=DIRECTION('center_axis',(0.,1.,0.));
#26857=DIRECTION('ref_axis',(0.689939110489398,0.,-0.723867407621795));
#26858=DIRECTION('',(0.,-1.,0.));
#26859=DIRECTION('center_axis',(0.,-1.,0.));
#26860=DIRECTION('ref_axis',(0.689939110489398,0.,-0.723867407621795));
#26861=DIRECTION('center_axis',(-0.0334572490706319,0.,-0.999440149526036));
#26862=DIRECTION('ref_axis',(-0.999440149526036,0.,0.0334572490706319));
#26863=DIRECTION('',(0.999440149526004,0.,-0.0334572490715974));
#26864=DIRECTION('',(0.,1.,0.));
#26865=DIRECTION('',(-0.999440149526004,0.,0.0334572490715974));
#26866=DIRECTION('center_axis',(0.,-1.,0.));
#26867=DIRECTION('ref_axis',(0.778520242143747,0.,0.627619496647803));
#26868=DIRECTION('center_axis',(0.,1.,0.));
#26869=DIRECTION('ref_axis',(0.778520242139959,0.,0.627619496652502));
#26870=DIRECTION('',(0.,-1.,0.));
#26871=DIRECTION('center_axis',(0.,-1.,0.));
#26872=DIRECTION('ref_axis',(0.778520242139959,0.,0.627619496652502));
#26873=DIRECTION('',(0.,1.,0.));
#26874=DIRECTION('center_axis',(0.,-1.,0.));
#26875=DIRECTION('ref_axis',(0.995256847821609,0.,-0.0972820994026908));
#26876=DIRECTION('center_axis',(0.,-1.,0.));
#26877=DIRECTION('ref_axis',(0.995256847821544,0.,-0.0972820994033552));
#26878=DIRECTION('',(0.,1.,0.));
#26879=DIRECTION('center_axis',(0.,1.,0.));
#26880=DIRECTION('ref_axis',(0.995256847821544,0.,-0.0972820994033552));
#26881=DIRECTION('center_axis',(0.,-1.,0.));
#26882=DIRECTION('ref_axis',(0.589552929365356,0.,-0.807729746559286));
#26883=DIRECTION('center_axis',(0.,1.,0.));
#26884=DIRECTION('ref_axis',(0.589552929372405,0.,-0.807729746554141));
#26885=DIRECTION('',(0.,-1.,0.));
#26886=DIRECTION('center_axis',(0.,-1.,0.));
#26887=DIRECTION('ref_axis',(0.589552929372405,0.,-0.807729746554141));
#26888=DIRECTION('center_axis',(-0.163624134736254,0.,-0.986522753174914));
#26889=DIRECTION('ref_axis',(-0.986522753174914,0.,0.163624134736254));
#26890=DIRECTION('',(0.986522753174779,0.,-0.163624134737066));
#26891=DIRECTION('',(0.,1.,0.));
#26892=DIRECTION('',(-0.986522753174779,0.,0.163624134737066));
#26893=DIRECTION('center_axis',(0.,-1.,0.));
#26894=DIRECTION('ref_axis',(0.853780676609419,0.,0.520632842076221));
#26895=DIRECTION('center_axis',(0.,1.,0.));
#26896=DIRECTION('ref_axis',(0.853780676602481,0.,0.520632842087598));
#26897=DIRECTION('',(0.,-1.,0.));
#26898=DIRECTION('center_axis',(0.,-1.,0.));
#26899=DIRECTION('ref_axis',(0.853780676602481,0.,0.520632842087598));
#26900=DIRECTION('',(0.,1.,0.));
#26901=DIRECTION('center_axis',(0.,-1.,0.));
#26902=DIRECTION('ref_axis',(0.974044425513625,0.,-0.22635692418354));
#26903=DIRECTION('center_axis',(0.,-1.,0.));
#26904=DIRECTION('ref_axis',(0.974044425513499,0.,-0.226356924184081));
#26905=DIRECTION('',(0.,1.,0.));
#26906=DIRECTION('center_axis',(0.,1.,0.));
#26907=DIRECTION('ref_axis',(0.974044425513499,0.,-0.226356924184081));
#26908=DIRECTION('center_axis',(0.,-1.,0.));
#26909=DIRECTION('ref_axis',(0.479079334165907,0.,-0.877771605587212));
#26910=DIRECTION('center_axis',(0.,1.,0.));
#26911=DIRECTION('ref_axis',(0.479079334179906,0.,-0.877771605579571));
#26912=DIRECTION('',(0.,-1.,0.));
#26913=DIRECTION('center_axis',(0.,-1.,0.));
#26914=DIRECTION('ref_axis',(0.479079334179906,0.,-0.877771605579571));
#26915=DIRECTION('center_axis',(-0.290991366091359,0.,-0.956725679001188));
#26916=DIRECTION('ref_axis',(-0.956725679001188,0.,0.290991366091359));
#26917=DIRECTION('',(0.956725679000994,0.,-0.290991366091996));
#26918=DIRECTION('',(0.,1.,0.));
#26919=DIRECTION('',(-0.956725679000994,0.,0.290991366091996));
#26920=DIRECTION('center_axis',(0.22635692418354,0.,0.974044425513625));
#26921=DIRECTION('ref_axis',(0.,-1.,0.));
#26922=DIRECTION('',(0.974044425513455,0.,-0.226356924184268));
#26923=DIRECTION('',(0.,-1.,0.));
#26924=DIRECTION('',(-0.974044425513455,0.,0.226356924184268));
#26925=DIRECTION('center_axis',(0.0972820994026909,0.,0.995256847821609));
#26926=DIRECTION('ref_axis',(0.,-1.,0.));
#26927=DIRECTION('',(0.995256847821521,0.,-0.0972820994035846));
#26928=DIRECTION('',(0.,-1.,0.));
#26929=DIRECTION('',(-0.995256847821521,0.,0.0972820994035846));
#26930=DIRECTION('center_axis',(-0.163624134736254,0.,0.986522753174914));
#26931=DIRECTION('ref_axis',(0.,1.,0.));
#26932=DIRECTION('',(0.986522753174779,0.,0.163624134737066));
#26933=DIRECTION('',(0.,-1.,0.));
#26934=DIRECTION('',(-0.986522753174779,0.,-0.163624134737066));
#26935=DIRECTION('center_axis',(-0.290991366091359,0.,0.956725679001188));
#26936=DIRECTION('ref_axis',(0.,1.,0.));
#26937=DIRECTION('',(0.956725679000994,0.,0.290991366091996));
#26938=DIRECTION('',(0.,-1.,0.));
#26939=DIRECTION('',(-0.956725679000994,0.,-0.290991366091996));
#26940=DIRECTION('center_axis',(0.,1.,0.));
#26941=DIRECTION('ref_axis',(-0.942641491092178,0.,-0.333806859233771));
#26942=DIRECTION('center_axis',(0.,-1.,0.));
#26943=DIRECTION('ref_axis',(-0.942641491092022,0.,-0.333806859234212));
#26944=DIRECTION('',(0.,-1.,0.));
#26945=DIRECTION('center_axis',(0.,1.,0.));
#26946=DIRECTION('ref_axis',(-0.942641491092022,0.,-0.333806859234212));
#26947=DIRECTION('center_axis',(0.,1.,0.));
#26948=DIRECTION('ref_axis',(-0.942641491092178,0.,-0.333806859233771));
#26949=DIRECTION('center_axis',(0.,1.,0.));
#26950=DIRECTION('ref_axis',(-0.942641491092022,0.,-0.333806859234212));
#26951=DIRECTION('center_axis',(0.,-1.,0.));
#26952=DIRECTION('ref_axis',(-0.942641491092022,0.,-0.333806859234212));
#26953=DIRECTION('center_axis',(0.,1.,0.));
#26954=DIRECTION('ref_axis',(1.,0.,0.));
#26955=DIRECTION('',(0.942641491091974,0.,-0.333806859234347));
#26956=DIRECTION('center_axis',(0.,-1.,0.));
#26957=DIRECTION('ref_axis',(0.942641491092032,0.,0.333806859234184));
#26958=DIRECTION('',(-0.942641491091975,0.,-0.333806859234346));
#26959=DIRECTION('center_axis',(0.,1.,0.));
#26960=DIRECTION('ref_axis',(-0.942641491092022,0.,-0.333806859234212));
#26961=DIRECTION('center_axis',(0.,1.,0.));
#26962=DIRECTION('ref_axis',(-0.942641491092022,0.,-0.333806859234212));
#26963=DIRECTION('center_axis',(0.,1.,0.));
#26964=DIRECTION('ref_axis',(-0.942641491092022,0.,-0.333806859234212));
#26965=DIRECTION('',(0.999440149526004,0.,0.0334572490715974));
#26966=DIRECTION('center_axis',(0.,1.,0.));
#26967=DIRECTION('ref_axis',(-0.942641491092022,0.,-0.333806859234212));
#26968=DIRECTION('center_axis',(0.,1.,0.));
#26969=DIRECTION('ref_axis',(-0.942641491092178,0.,-0.333806859233771));
#26970=DIRECTION('center_axis',(0.,-1.,0.));
#26971=DIRECTION('ref_axis',(-0.942641491092022,0.,-0.333806859234212));
#26972=DIRECTION('',(0.,-1.,0.));
#26973=DIRECTION('center_axis',(0.,1.,0.));
#26974=DIRECTION('ref_axis',(-0.942641491092178,0.,-0.333806859233771));
#26975=DIRECTION('',(0.,1.,0.));
#26976=DIRECTION('center_axis',(0.,-1.,0.));
#26977=DIRECTION('ref_axis',(-0.942641491092022,0.,-0.333806859234212));
#26978=DIRECTION('center_axis',(-0.0334572490706319,0.,0.999440149526036));
#26979=DIRECTION('ref_axis',(0.,1.,0.));
#26980=DIRECTION('',(-0.999440149526004,0.,-0.0334572490715974));
#26981=DIRECTION('center_axis',(0.,1.,0.));
#26982=DIRECTION('ref_axis',(-0.942641491092178,0.,-0.333806859233771));
#26983=DIRECTION('center_axis',(0.,-1.,0.));
#26984=DIRECTION('ref_axis',(-0.942641491092022,0.,-0.333806859234212));
#26985=DIRECTION('center_axis',(-0.333806859233773,0.,-0.942641491092178));
#26986=DIRECTION('ref_axis',(-0.942641491092178,0.,0.333806859233773));
#26987=DIRECTION('',(-0.942641491091974,0.,0.333806859234347));
#26988=DIRECTION('',(0.,1.,0.));
#26989=DIRECTION('center_axis',(0.,1.,0.));
#26990=DIRECTION('ref_axis',(0.942641491092178,0.,0.333806859233771));
#26991=DIRECTION('center_axis',(0.,1.,0.));
#26992=DIRECTION('ref_axis',(0.942641491092032,0.,0.333806859234184));
#26993=DIRECTION('',(0.,1.,0.));
#26994=DIRECTION('center_axis',(-0.333806859233772,0.,0.942641491092178));
#26995=DIRECTION('ref_axis',(0.,1.,0.));
#26996=DIRECTION('',(0.942641491091975,0.,0.333806859234346));
#26997=DIRECTION('center_axis',(0.,1.,0.));
#26998=DIRECTION('ref_axis',(-0.942641491092178,0.,-0.333806859233771));
#26999=DIRECTION('center_axis',(0.,-1.,0.));
#27000=DIRECTION('ref_axis',(-0.942641491092022,0.,-0.333806859234212));
#27001=DIRECTION('center_axis',(0.,1.,0.));
#27002=DIRECTION('ref_axis',(1.,0.,0.));
#32956=CARTESIAN_POINT('',(0.,0.,0.));
#32957=CARTESIAN_POINT('Origin',(0.0126992616256242,-0.008,0.00360121565085291));
#32958=CARTESIAN_POINT('',(0.0126265137841014,-0.008,0.00384039707060321));
#32959=CARTESIAN_POINT('',(0.0129397779442914,-0.008,0.00366942049272513));
#32960=CARTESIAN_POINT('Origin',(0.0126992616256341,-0.00799999999999,0.00360121565086291));
#32961=CARTESIAN_POINT('',(0.0129397779442914,-0.024,0.00366942049272513));
#32962=CARTESIAN_POINT('',(0.0129397779443013,-0.00799999999999,0.00366942049273513));
#32963=CARTESIAN_POINT('',(0.0126265137841014,-0.024,0.00384039707060321));
#32964=CARTESIAN_POINT('Origin',(0.0126992616256341,-0.02400000000001,0.00360121565086291));
#32965=CARTESIAN_POINT('',(0.0126265137841114,-0.00799999999999,0.00384039707061321));
#32966=CARTESIAN_POINT('Origin',(-4.44089209850063E-17,-0.008,6.72997231505748E-33));
#32967=CARTESIAN_POINT('',(0.0130408866654485,-0.008,0.0032920776082785));
#32968=CARTESIAN_POINT('Origin',(-4.44089209850063E-17,-0.00799999999999,
6.72997231505748E-33));
#32969=CARTESIAN_POINT('',(0.0130408866654485,-0.024,0.0032920776082785));
#32970=CARTESIAN_POINT('',(0.0130408866654585,-0.00799999999999,0.0032920776082885));
#32971=CARTESIAN_POINT('Origin',(-4.44089209850063E-17,-0.02400000000001,
6.72997231505748E-33));
#32972=CARTESIAN_POINT('Origin',(0.0127984910025219,-0.008,0.00323088657466738));
#32973=CARTESIAN_POINT('',(0.0128550802335678,-0.008,0.00298737546828897));
#32974=CARTESIAN_POINT('Origin',(0.0127984910025319,-0.00799999999999,0.00323088657467738));
#32975=CARTESIAN_POINT('',(0.0128550802335678,-0.024,0.00298737546828897));
#32976=CARTESIAN_POINT('',(0.0128550802335778,-0.00799999999999,0.00298737546829897));
#32977=CARTESIAN_POINT('Origin',(0.0127984910025319,-0.02400000000001,0.00323088657467738));
#32978=CARTESIAN_POINT('Origin',(0.0126625775316771,-0.008,0.00294264001438602));
#32979=CARTESIAN_POINT('',(0.0126625775316771,-0.008,0.00294264001438602));
#32980=CARTESIAN_POINT('',(0.0125348531511851,-0.00799999999999,0.00291295831081412));
#32981=CARTESIAN_POINT('',(0.0126625775316771,-0.024,0.00294264001438602));
#32982=CARTESIAN_POINT('',(0.0126625775316871,-0.016,0.00294264001439602));
#32983=CARTESIAN_POINT('',(0.0125348531511851,-0.02400000000001,0.00291295831081412));
#32984=CARTESIAN_POINT('Origin',(0.0130606706482359,-0.008,0.00191282048773811));
#32985=CARTESIAN_POINT('',(0.0130197646145518,-0.008,0.00215945117603184));
#32986=CARTESIAN_POINT('',(0.0133080318347555,-0.008,0.00194904814849073));
#32987=CARTESIAN_POINT('Origin',(0.0130606706482459,-0.00799999999999,0.00191282048774811));
#32988=CARTESIAN_POINT('',(0.0133080318347555,-0.024,0.00194904814849073));
#32989=CARTESIAN_POINT('',(0.0133080318347655,-0.00799999999999,0.00194904814850073));
#32990=CARTESIAN_POINT('',(0.0130197646145518,-0.024,0.00215945117603184));
#32991=CARTESIAN_POINT('Origin',(0.0130606706482459,-0.02400000000001,0.00191282048774811));
#32992=CARTESIAN_POINT('',(0.0130197646145618,-0.00799999999999,0.00215945117604184));
#32993=CARTESIAN_POINT('Origin',(-4.44089209850063E-17,-0.008,6.72997231505748E-33));
#32994=CARTESIAN_POINT('',(0.0133590224269186,-0.008,0.00156173614835727));
#32995=CARTESIAN_POINT('Origin',(-4.44089209850063E-17,-0.00799999999999,
6.72997231505748E-33));
#32996=CARTESIAN_POINT('',(0.0133590224269186,-0.024,0.00156173614835727));
#32997=CARTESIAN_POINT('',(0.0133590224269286,-0.00799999999999,0.00156173614836727));
#32998=CARTESIAN_POINT('Origin',(-4.44089209850063E-17,-0.02400000000001,
6.72997231505748E-33));
#32999=CARTESIAN_POINT('Origin',(0.0131107134598755,-0.008,0.00153270759541383));
#33000=CARTESIAN_POINT('',(0.0131350339847262,-0.008,0.00128389338345843));
#33001=CARTESIAN_POINT('Origin',(0.0131107134598855,-0.00799999999999,0.00153270759542383));
#33002=CARTESIAN_POINT('',(0.0131350339847262,-0.024,0.00128389338345843));
#33003=CARTESIAN_POINT('',(0.0131350339847362,-0.00799999999999,0.00128389338346843));
#33004=CARTESIAN_POINT('Origin',(0.0131107134598855,-0.02400000000001,0.00153270759542383));
#33005=CARTESIAN_POINT('Origin',(0.0129383390216809,-0.008,0.00126466729223498));
#33006=CARTESIAN_POINT('',(0.0129383390216809,-0.008,0.00126466729223498));
#33007=CARTESIAN_POINT('',(0.0129458744527519,-0.00799999999999,0.00126540384839641));
#33008=CARTESIAN_POINT('',(0.0129383390216809,-0.024,0.00126466729223498));
#33009=CARTESIAN_POINT('',(0.0129383390216909,-0.016,0.00126466729224498));
#33010=CARTESIAN_POINT('',(0.0129458744527519,-0.02400000000001,0.00126540384839641));
#33011=CARTESIAN_POINT('Origin',(0.0131986079749541,-0.008,0.00019169643574408));
#33012=CARTESIAN_POINT('',(0.0131902436626865,-0.008,0.000441556473125589));
#33013=CARTESIAN_POINT('',(0.0134485816108434,-0.008,0.000195327050057415));
#33014=CARTESIAN_POINT('Origin',(0.0131986079749641,-0.00799999999999,0.00019169643575408));
#33015=CARTESIAN_POINT('',(0.0134485816108434,-0.024,0.000195327050057415));
#33016=CARTESIAN_POINT('',(0.0134485816108534,-0.00799999999999,0.000195327050067415));
#33017=CARTESIAN_POINT('',(0.0131902436626865,-0.024,0.000441556473125589));
#33018=CARTESIAN_POINT('Origin',(0.0131986079749641,-0.02400000000001,0.00019169643575408));
#33019=CARTESIAN_POINT('',(0.0131902436626965,-0.00799999999999,0.000441556473135589));
#33020=CARTESIAN_POINT('Origin',(-4.44089209850063E-17,-0.008,6.72997231505748E-33));
#33021=CARTESIAN_POINT('',(0.0134485816108434,-0.008,-0.000195327050057413));
#33022=CARTESIAN_POINT('Origin',(-4.44089209850063E-17,-0.00799999999999,
6.72997231505748E-33));
#33023=CARTESIAN_POINT('',(0.0134485816108434,-0.024,-0.000195327050057413));
#33024=CARTESIAN_POINT('',(0.0134485816108534,-0.00799999999999,-0.000195327050067413));
#33025=CARTESIAN_POINT('Origin',(-4.44089209850063E-17,-0.02400000000001,
6.72997231505748E-33));
#33026=CARTESIAN_POINT('Origin',(0.0131986079749541,-0.008,-0.000191696435744079));
#33027=CARTESIAN_POINT('',(0.0131902436626865,-0.008,-0.000441556473125588));
#33028=CARTESIAN_POINT('Origin',(0.0131986079749641,-0.00799999999999,-0.000191696435754079));
#33029=CARTESIAN_POINT('',(0.0131902436626865,-0.024,-0.000441556473125588));
#33030=CARTESIAN_POINT('',(0.0131902436626965,-0.00799999999999,-0.000441556473135588));
#33031=CARTESIAN_POINT('Origin',(0.0131986079749641,-0.02400000000001,-0.000191696435754079));
#33032=CARTESIAN_POINT('Origin',(0.0129927219438385,-0.008,-0.000434944237918216));
#33033=CARTESIAN_POINT('',(0.0129927219438385,-0.008,-0.000434944237918216));
#33034=CARTESIAN_POINT('',(0.0130276266077339,-0.00799999999999,-0.000436112706129034));
#33035=CARTESIAN_POINT('',(0.0129927219438385,-0.024,-0.000434944237918216));
#33036=CARTESIAN_POINT('',(0.0129927219438485,-0.016,-0.000434944237928215));
#33037=CARTESIAN_POINT('',(0.0130276266077339,-0.02400000000001,-0.000436112706129034));
#33038=CARTESIAN_POINT('Origin',(0.0131107134598755,-0.008,-0.00153270759541383));
#33039=CARTESIAN_POINT('',(0.0131350339847262,-0.008,-0.00128389338345843));
#33040=CARTESIAN_POINT('',(0.0133590224269186,-0.008,-0.00156173614835727));
#33041=CARTESIAN_POINT('Origin',(0.0131107134598855,-0.00799999999999,-0.00153270759542383));
#33042=CARTESIAN_POINT('',(0.0133590224269186,-0.024,-0.00156173614835727));
#33043=CARTESIAN_POINT('',(0.0133590224269286,-0.00799999999999,-0.00156173614836727));
#33044=CARTESIAN_POINT('',(0.0131350339847262,-0.024,-0.00128389338345843));
#33045=CARTESIAN_POINT('Origin',(0.0131107134598855,-0.02400000000001,-0.00153270759542383));
#33046=CARTESIAN_POINT('',(0.0131350339847362,-0.00799999999999,-0.00128389338346843));
#33047=CARTESIAN_POINT('Origin',(-4.44089209850063E-17,-0.008,6.72997231505748E-33));
#33048=CARTESIAN_POINT('',(0.0133080318347555,-0.008,-0.00194904814849073));
#33049=CARTESIAN_POINT('Origin',(-4.44089209850063E-17,-0.00799999999999,
6.72997231505748E-33));
#33050=CARTESIAN_POINT('',(0.0133080318347555,-0.024,-0.00194904814849073));
#33051=CARTESIAN_POINT('',(0.0133080318347655,-0.00799999999999,-0.00194904814850073));
#33052=CARTESIAN_POINT('Origin',(-4.44089209850063E-17,-0.02400000000001,
6.72997231505748E-33));
#33053=CARTESIAN_POINT('Origin',(0.0130606706482359,-0.008,-0.00191282048773811));
#33054=CARTESIAN_POINT('',(0.0130197646145518,-0.008,-0.00215945117603184));
#33055=CARTESIAN_POINT('Origin',(0.0130606706482459,-0.00799999999999,-0.00191282048774811));
#33056=CARTESIAN_POINT('',(0.0130197646145518,-0.024,-0.00215945117603184));
#33057=CARTESIAN_POINT('',(0.0130197646145618,-0.00799999999999,-0.00215945117604184));
#33058=CARTESIAN_POINT('Origin',(0.0130606706482459,-0.02400000000001,-0.00191282048774811));
#33059=CARTESIAN_POINT('Origin',(0.0128247957912738,-0.008,-0.00212711375157131));
#33060=CARTESIAN_POINT('',(0.0128247957912738,-0.008,-0.00212711375157131));
#33061=CARTESIAN_POINT('',(0.0127759261415696,-0.00799999999999,-0.00211900825769013));
#33062=CARTESIAN_POINT('',(0.0128247957912738,-0.024,-0.00212711375157131));
#33063=CARTESIAN_POINT('',(0.0128247957912839,-0.016,-0.00212711375158131));
#33064=CARTESIAN_POINT('',(0.0127759261415696,-0.02400000000001,-0.00211900825769013));
#33065=CARTESIAN_POINT('Origin',(0.0127984910025219,-0.008,-0.00323088657466738));
#33066=CARTESIAN_POINT('',(0.0128550802335678,-0.008,-0.00298737546828897));
#33067=CARTESIAN_POINT('',(0.0130408866654485,-0.008,-0.0032920776082785));
#33068=CARTESIAN_POINT('Origin',(0.0127984910025319,-0.00799999999999,-0.00323088657467738));
#33069=CARTESIAN_POINT('',(0.0130408866654485,-0.024,-0.0032920776082785));
#33070=CARTESIAN_POINT('',(0.0130408866654585,-0.00799999999999,-0.0032920776082885));
#33071=CARTESIAN_POINT('',(0.0128550802335678,-0.024,-0.00298737546828897));
#33072=CARTESIAN_POINT('Origin',(0.0127984910025319,-0.02400000000001,-0.00323088657467738));
#33073=CARTESIAN_POINT('',(0.0128550802335778,-0.00799999999999,-0.00298737546829897));
#33074=CARTESIAN_POINT('Origin',(-4.44089209850063E-17,-0.008,6.72997231505748E-33));
#33075=CARTESIAN_POINT('',(0.0129397779442914,-0.008,-0.00366942049272513));
#33076=CARTESIAN_POINT('Origin',(-4.44089209850063E-17,-0.00799999999999,
6.72997231505748E-33));
#33077=CARTESIAN_POINT('',(0.0129397779442914,-0.024,-0.00366942049272513));
#33078=CARTESIAN_POINT('',(0.0129397779443013,-0.00799999999999,-0.00366942049273513));
#33079=CARTESIAN_POINT('Origin',(-4.44089209850063E-17,-0.02400000000001,
6.72997231505748E-33));
#33080=CARTESIAN_POINT('Origin',(0.0126992616256242,-0.008,-0.00360121565085291));
#33081=CARTESIAN_POINT('',(0.0126265137841014,-0.008,-0.00384039707060321));
#33082=CARTESIAN_POINT('Origin',(0.0126992616256341,-0.00799999999999,-0.00360121565086291));
#33083=CARTESIAN_POINT('',(0.0126265137841014,-0.024,-0.00384039707060321));
#33084=CARTESIAN_POINT('',(0.0126265137841114,-0.00799999999999,-0.00384039707061321));
#33085=CARTESIAN_POINT('Origin',(0.0126992616256341,-0.02400000000001,-0.00360121565086291));
#33086=CARTESIAN_POINT('Origin',(0.0124374338270155,-0.008,-0.00378288775918766));
#33087=CARTESIAN_POINT('',(0.0124374338270155,-0.008,-0.00378288775918766));
#33088=CARTESIAN_POINT('',(0.0122036407116943,-0.00799999999999,-0.00371177878877263));
#33089=CARTESIAN_POINT('',(0.0124374338270155,-0.024,-0.00378288775918766));
#33090=CARTESIAN_POINT('',(0.0124374338270255,-0.016,-0.00378288775919766));
#33091=CARTESIAN_POINT('',(0.0122036407116943,-0.02400000000001,-0.00371177878877263));
#33092=CARTESIAN_POINT('Origin',(0.0131008975231583,-0.008,-0.00304450063026861));
#33093=CARTESIAN_POINT('',(0.0126625775316771,-0.024,-0.00294264001438602));
#33094=CARTESIAN_POINT('',(0.0127540131469256,-0.02400000000001,-0.00296388861875541));
#33095=CARTESIAN_POINT('',(0.0126625775316771,-0.008,-0.00294264001438602));
#33096=CARTESIAN_POINT('',(0.0126625775316871,-0.016,-0.00294264001439602));
#33097=CARTESIAN_POINT('',(0.0127540131469256,-0.00799999999999,-0.00296388861875541));
#33098=CARTESIAN_POINT('Origin',(0.0133862046032006,-0.008,-0.00130844423696619));
#33099=CARTESIAN_POINT('',(0.0129383390216809,-0.024,-0.00126466729223498));
#33100=CARTESIAN_POINT('',(0.0131698072435117,-0.02400000000001,-0.00128729232076201));
#33101=CARTESIAN_POINT('',(0.0129383390216809,-0.008,-0.00126466729223498));
#33102=CARTESIAN_POINT('',(0.0129383390216909,-0.016,-0.00126466729224498));
#33103=CARTESIAN_POINT('',(0.0131698072435117,-0.00799999999999,-0.00128729232076201));
#33104=CARTESIAN_POINT('Origin',(0.0132687310302026,-0.008,0.00220074461220262));
#33105=CARTESIAN_POINT('',(0.0128247957912738,-0.024,0.00212711375157131));
#33106=CARTESIAN_POINT('',(0.0129978937610339,-0.02400000000001,0.00215582368800579));
#33107=CARTESIAN_POINT('',(0.0128247957912738,-0.008,0.00212711375157131));
#33108=CARTESIAN_POINT('',(0.0128247957912839,-0.016,0.0021271137515813));
#33109=CARTESIAN_POINT('',(0.0129978937610339,-0.00799999999999,0.00215582368800579));
#33110=CARTESIAN_POINT('Origin',(0.012867960382566,-0.008,0.00391383387392877));
#33111=CARTESIAN_POINT('',(0.0124374338270155,-0.024,0.00378288775918766));
#33112=CARTESIAN_POINT('',(0.0124189039894696,-0.02400000000001,0.00377725184614318));
#33113=CARTESIAN_POINT('',(0.0124374338270155,-0.008,0.00378288775918766));
#33114=CARTESIAN_POINT('',(0.0124374338270255,-0.016,0.00378288775919766));
#33115=CARTESIAN_POINT('',(0.0124189039894696,-0.00799999999999,0.00377725184614318));
#33116=CARTESIAN_POINT('Origin',(-4.44089209850063E-17,-0.016,6.72997231505748E-33));
#33117=CARTESIAN_POINT('',(0.0122543393841983,-0.008,-0.00433948917003902));
#33118=CARTESIAN_POINT('Origin',(-4.44089209850063E-17,-0.00799999999999,
6.72997231505748E-33));
#33119=CARTESIAN_POINT('',(0.0122543393841983,-0.024,-0.00433948917003902));
#33120=CARTESIAN_POINT('',(0.0122543393842083,-0.016,-0.00433948917004902));
#33121=CARTESIAN_POINT('Origin',(-4.44089209850063E-17,-0.02400000000001,
6.72997231505748E-33));
#33122=CARTESIAN_POINT('Origin',(-4.44089209850063E-17,-0.016,6.72997231505748E-33));
#33123=CARTESIAN_POINT('Origin',(-4.44089209850063E-17,-0.02400000000001,
6.72997231505748E-33));
#33124=CARTESIAN_POINT('Origin',(-4.44089209850063E-17,-0.00799999999999,
6.72997231505748E-33));
#33125=CARTESIAN_POINT('Origin',(0.0130771696920991,-0.024,1.11022302462517E-18));
#33126=CARTESIAN_POINT('',(0.0131027167261813,-0.024,-0.00463991534334942));
#33127=CARTESIAN_POINT('',(0.0131027167261912,-0.02400000000001,-0.00463991534335942));
#33128=CARTESIAN_POINT('',(0.0131027167261813,-0.024,0.00463991534334942));
#33129=CARTESIAN_POINT('Origin',(-4.44089209850063E-17,-0.02400000000001,
6.72997231505748E-33));
#33130=CARTESIAN_POINT('',(0.0122543393841983,-0.024,0.00433948917003903));
#33131=CARTESIAN_POINT('',(0.0122543393842083,-0.02400000000001,0.00433948917004903));
#33132=CARTESIAN_POINT('Origin',(-4.44089209850063E-17,-0.02400000000001,
6.72997231505748E-33));
#33133=CARTESIAN_POINT('Origin',(-4.44089209850063E-17,-0.02400000000001,
6.72997231505748E-33));
#33134=CARTESIAN_POINT('',(0.0129927219438385,-0.024,0.000434944237918216));
#33135=CARTESIAN_POINT('Origin',(-4.44089209850063E-17,-0.02400000000001,
6.72997231505748E-33));
#33136=CARTESIAN_POINT('',(0.0132525006413773,-0.02400000000001,0.000443640587169928));
#33137=CARTESIAN_POINT('Origin',(-4.44089209850063E-17,-0.02400000000001,
6.72997231505748E-33));
#33138=CARTESIAN_POINT('Origin',(-4.44089209850063E-17,-0.016,6.72997231505748E-33));
#33139=CARTESIAN_POINT('',(0.0129927219438385,-0.008,0.000434944237918216));
#33140=CARTESIAN_POINT('Origin',(-4.44089209850063E-17,-0.00799999999999,
6.72997231505748E-33));
#33141=CARTESIAN_POINT('',(0.0129927219438485,-0.016,0.000434944237928217));
#33142=CARTESIAN_POINT('Origin',(-4.44089209850063E-17,-0.016,6.72997231505748E-33));
#33143=CARTESIAN_POINT('',(0.0122543393841983,-0.008,0.00433948917003903));
#33144=CARTESIAN_POINT('',(0.0122543393842083,-0.016,0.00433948917004903));
#33145=CARTESIAN_POINT('Origin',(-4.44089209850063E-17,-0.00799999999999,
6.72997231505748E-33));
#33146=CARTESIAN_POINT('Origin',(0.0134424700111252,-0.008,0.00045));
#33147=CARTESIAN_POINT('',(0.0132525006413773,-0.00799999999999,0.000443640587169928));
#33148=CARTESIAN_POINT('Origin',(-4.44089209850063E-17,-0.016,6.72997231505748E-33));
#33149=CARTESIAN_POINT('Origin',(-4.44089209850063E-17,-0.00799999999999,
6.72997231505748E-33));
#33150=CARTESIAN_POINT('Origin',(0.0131027167261813,-0.016,-0.00463991534334942));
#33151=CARTESIAN_POINT('',(0.0131027167261813,-0.008,-0.00463991534334942));
#33152=CARTESIAN_POINT('',(0.0131027167261912,-0.00799999999999,-0.00463991534335942));
#33153=CARTESIAN_POINT('',(0.0131027167261912,-0.016,-0.00463991534335942));
#33154=CARTESIAN_POINT('Origin',(-4.44089209850063E-17,-0.016,6.72997231505748E-33));
#33155=CARTESIAN_POINT('',(0.0131027167261813,-0.008,0.00463991534334942));
#33156=CARTESIAN_POINT('Origin',(-4.44089209850063E-17,-0.00799999999999,
6.72997231505748E-33));
#33157=CARTESIAN_POINT('',(0.0131027167261912,-0.016,0.00463991534335942));
#33158=CARTESIAN_POINT('Origin',(0.0122543393841983,-0.016,0.00433948917003903));
#33159=CARTESIAN_POINT('',(0.0122543393842083,-0.00799999999999,0.00433948917004903));
#33160=CARTESIAN_POINT('Origin',(-4.44089209850063E-17,-0.016,6.72997231505748E-33));
#33161=CARTESIAN_POINT('Origin',(-4.44089209850063E-17,-0.00799999999999,
6.72997231505748E-33));
#33162=CARTESIAN_POINT('Origin',(0.0130771696920991,-0.008,1.11022302462517E-18));
#34830=UNCERTAINTY_MEASURE_WITH_UNIT(LENGTH_MEASURE(1.E-5),#34877,
'DISTANCE_ACCURACY_VALUE',
'Maximum model space distance between geometric entities at asserted c
onnectivities');
#34841=UNCERTAINTY_MEASURE_WITH_UNIT(LENGTH_MEASURE(1.E-5),#34877,
'DISTANCE_ACCURACY_VALUE',
'Maximum model space distance between geometric entities at asserted c
onnectivities');
#34865=(
GEOMETRIC_REPRESENTATION_CONTEXT(3)
GLOBAL_UNCERTAINTY_ASSIGNED_CONTEXT((#34830))
GLOBAL_UNIT_ASSIGNED_CONTEXT((#34877,#34878,#34879))
REPRESENTATION_CONTEXT('','3D')
);
#34876=(
GEOMETRIC_REPRESENTATION_CONTEXT(3)
GLOBAL_UNCERTAINTY_ASSIGNED_CONTEXT((#34841))
GLOBAL_UNIT_ASSIGNED_CONTEXT((#34877,#34878,#34879))
REPRESENTATION_CONTEXT('','3D')
);
#34877=(
LENGTH_UNIT()
NAMED_UNIT(*)
SI_UNIT($,.METRE.)
);
#34878=(
NAMED_UNIT(*)
PLANE_ANGLE_UNIT()
SI_UNIT($,.RADIAN.)
);
#34879=(
NAMED_UNIT(*)
SI_UNIT($,.STERADIAN.)
SOLID_ANGLE_UNIT()
);
#34903=SHAPE_DEFINITION_REPRESENTATION(#34937,#35007);
#34937=PRODUCT_DEFINITION_SHAPE('',$,#35042);
#35007=SHAPE_REPRESENTATION('',(#21667),#34865);
#35018=PRODUCT_DEFINITION_CONTEXT('part definition',#35122,'design');
#35042=PRODUCT_DEFINITION('Motor Stator Face 5','Motor Stator Face 5',#35076,
#35018);
#35076=PRODUCT_DEFINITION_FORMATION('',$,#35147);
#35122=APPLICATION_CONTEXT('Managed model based 3d engineering');
#35123=PRODUCT_CONTEXT('part definition',#35122,'mechanical');
#35147=PRODUCT('Motor Stator Face 5','Motor Stator Face 5',
'LEGAL AND USAGE DISCLAIMER: this Data/Model is provided \X2\201C\X0\A
S IS\X2\201D\X0\ for informational and representational only. It is a 
geometric approximation and is NOT engineered, certified, or guarantee
d for dimensional accuracy, exact tolerances, or production-level prec
ision. Vendor disclaims all implied warranties including fitness for a
 particular purpose. DO NOT USE FOR DIRECT PHYSICAL MANUFACTURING, AUT
OMATED PRODUCTION, OR SAFETY-CRITICAL SYSTEMS without independent engi
neering verification and resolution of any design discrepancies.',(#35123));
#35165=PRESENTATION_STYLE_ASSIGNMENT((#35174));
#35174=SURFACE_STYLE_USAGE(.BOTH.,#35183);
#35183=SURFACE_SIDE_STYLE('',(#35192));
#35192=SURFACE_STYLE_FILL_AREA(#35201);
#35201=FILL_AREA_STYLE('Paint - Metallic (Blue)',(#35210));
#35210=FILL_AREA_STYLE_COLOUR('Paint - Metallic (Blue)',#35219);
#35219=COLOUR_RGB('Paint - Metallic (Blue)',0.188235294117647,0.231372549019608,
0.588235294117647);
ENDSEC;
END-ISO-10303-21;
